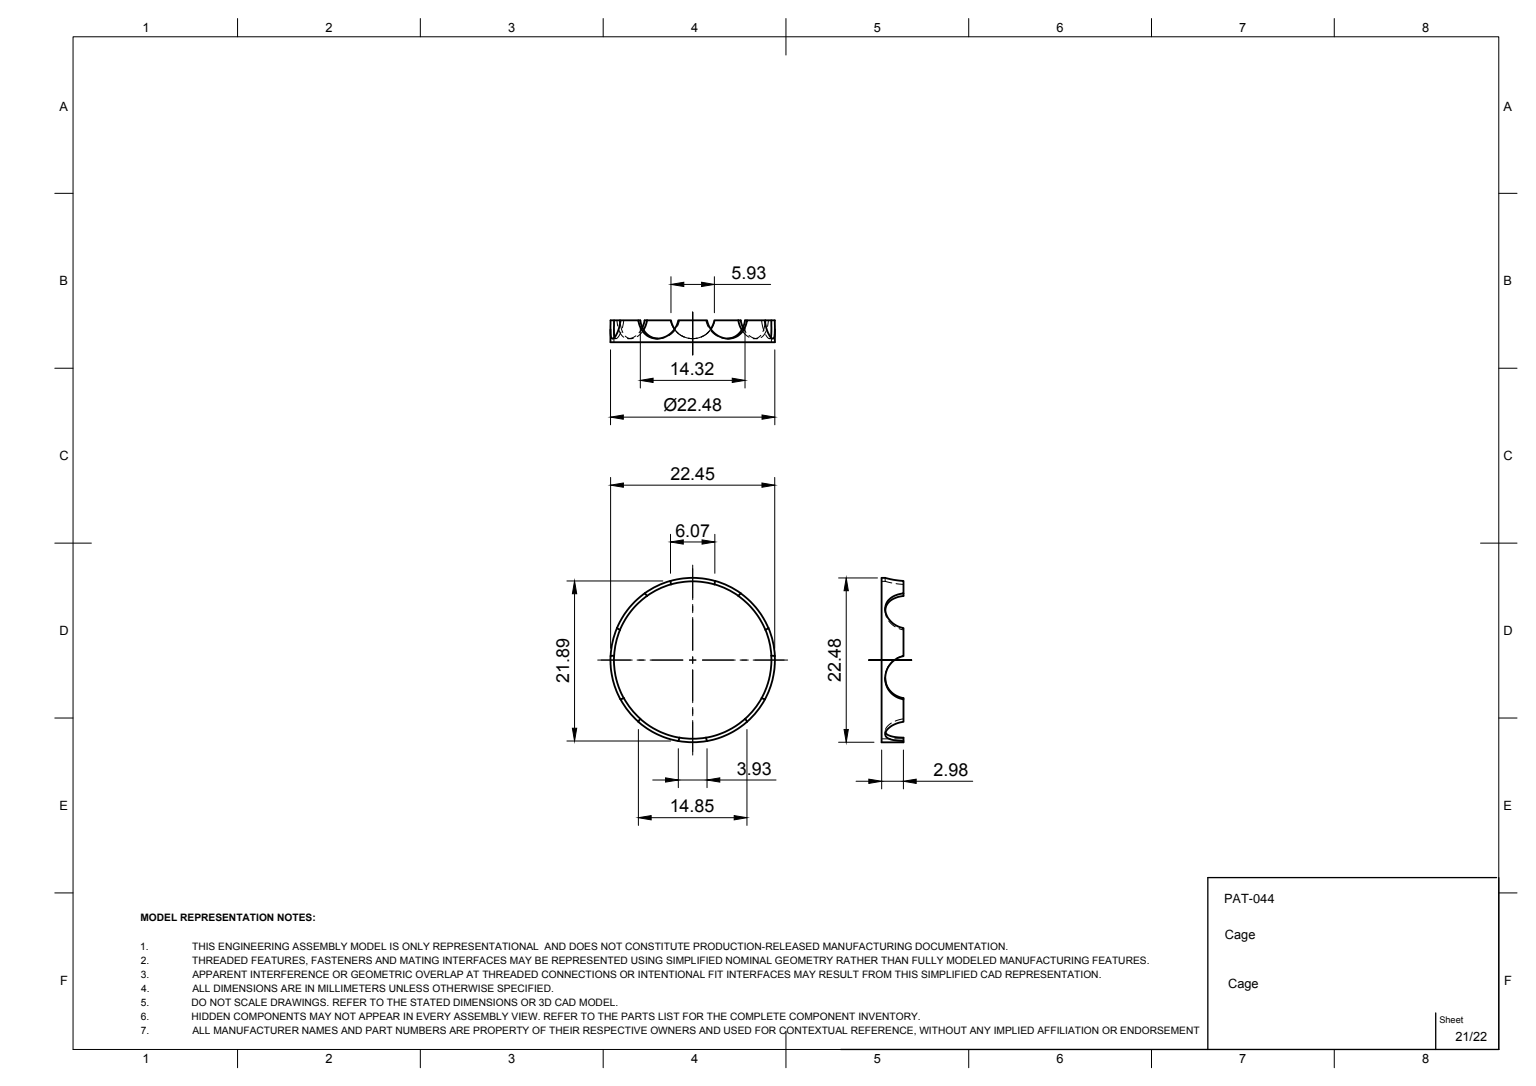
ISO-10303-21;
HEADER;
/* Generated by software containing ST-Developer
 * from STEP Tools, Inc. (www.steptools.com) 
 */

FILE_DESCRIPTION(
/* description */ ('Four-wheel beam trolley'),
/* implementation_level */ '2;1');

FILE_NAME(
/* name */ 'Cage.step',
/* time_stamp */ '2026-10-29T16:22:06-07:00',
/* author */ (''),
/* organization */ (''),
/* preprocessor_version */ 'ST-DEVELOPER v20.2',
/* originating_system */ 'Autodesk Translation Framework v15.17.0.0',
/* authorisation */ '');

FILE_SCHEMA (('AUTOMOTIVE_DESIGN { 1 0 10303 214 3 1 1 }'));
ENDSEC;

DATA;
#10=MECHANICAL_DESIGN_GEOMETRIC_PRESENTATION_REPRESENTATION('',(#298),#4777);
#11=B_SPLINE_CURVE_WITH_KNOTS('',3,(#4287,#4288,#4289,#4290,#4291,#4292,
#4293,#4294,#4295,#4296,#4297,#4298,#4299,#4300,#4301,#4302,#4303,#4304,
#4305,#4306,#4307,#4308),.UNSPECIFIED.,.F.,.F.,(4,2,2,2,2,2,2,2,2,2,4),
(0.0591825211272536,0.157966726598481,0.236950089897721,0.315933453196962,
0.391576304923761,0.46721915665056,0.54286200837736,0.618504860104159,0.697488223403399,
0.77647158670264,0.875255792173867),.UNSPECIFIED.);
#12=B_SPLINE_CURVE_WITH_KNOTS('',3,(#4312,#4313,#4314,#4315,#4316,#4317,
#4318,#4319,#4320,#4321,#4322,#4323,#4324,#4325,#4326,#4327,#4328,#4329,
#4330,#4331,#4332,#4333),.UNSPECIFIED.,.F.,.F.,(4,2,2,2,2,2,2,2,2,2,4),
(0.0581119756758434,0.106553146291161,0.213106292582322,0.30849933801665,
0.386091982889075,0.4636846277615,0.541277272633925,0.61886991750635,0.714262962940678,
0.820816109231839,0.869257279847157),.UNSPECIFIED.);
#13=B_SPLINE_CURVE_WITH_KNOTS('',3,(#4339,#4340,#4341,#4342,#4343,#4344,
#4345,#4346,#4347,#4348,#4349,#4350,#4351,#4352,#4353,#4354,#4355,#4356,
#4357,#4358,#4359,#4360),.UNSPECIFIED.,.F.,.F.,(4,2,2,2,2,2,2,2,2,2,4),
(0.0581119756758434,0.106553146291161,0.213106292582322,0.30849933801665,
0.386091982889075,0.4636846277615,0.541277272633925,0.61886991750635,0.714262962940679,
0.820816109231839,0.869257279847157),.UNSPECIFIED.);
#14=B_SPLINE_CURVE_WITH_KNOTS('',3,(#4364,#4365,#4366,#4367,#4368,#4369,
#4370,#4371,#4372,#4373,#4374,#4375,#4376,#4377,#4378,#4379,#4380,#4381,
#4382,#4383,#4384,#4385),.UNSPECIFIED.,.F.,.F.,(4,2,2,2,2,2,2,2,2,2,4),
(0.0581119756758433,0.106553146291161,0.213106292582322,0.308499338016649,
0.386091982889075,0.4636846277615,0.541277272633925,0.61886991750635,0.714262962940678,
0.820816109231839,0.869257279847157),.UNSPECIFIED.);
#15=B_SPLINE_CURVE_WITH_KNOTS('',3,(#4394,#4395,#4396,#4397,#4398,#4399,
#4400,#4401,#4402,#4403,#4404,#4405,#4406,#4407,#4408,#4409,#4410,#4411,
#4412,#4413,#4414,#4415),.UNSPECIFIED.,.F.,.F.,(4,2,2,2,2,2,2,2,2,2,4),
(0.0581119756758433,0.106553146291161,0.213106292582322,0.30849933801665,
0.386091982889075,0.4636846277615,0.541277272633925,0.61886991750635,0.714262962940678,
0.820816109231839,0.869257279847157),.UNSPECIFIED.);
#16=B_SPLINE_CURVE_WITH_KNOTS('',3,(#4419,#4420,#4421,#4422,#4423,#4424,
#4425,#4426,#4427,#4428,#4429,#4430,#4431,#4432,#4433,#4434,#4435,#4436,
#4437,#4438,#4439,#4440),.UNSPECIFIED.,.F.,.F.,(4,2,2,2,2,2,2,2,2,2,4),
(0.0581119756758434,0.106553146291161,0.213106292582322,0.30849933801665,
0.386091982889075,0.4636846277615,0.541277272633925,0.61886991750635,0.714262962940678,
0.820816109231839,0.869257279847157),.UNSPECIFIED.);
#17=B_SPLINE_CURVE_WITH_KNOTS('',3,(#4444,#4445,#4446,#4447,#4448,#4449,
#4450,#4451,#4452,#4453,#4454,#4455,#4456,#4457,#4458,#4459,#4460,#4461,
#4462,#4463,#4464,#4465),.UNSPECIFIED.,.F.,.F.,(4,2,2,2,2,2,2,2,2,2,4),
(0.0581119756758434,0.106553146291161,0.213106292582322,0.30849933801665,
0.386091982889075,0.4636846277615,0.541277272633925,0.61886991750635,0.714262962940678,
0.820816109231839,0.869257279847157),.UNSPECIFIED.);
#18=B_SPLINE_CURVE_WITH_KNOTS('',3,(#4469,#4470,#4471,#4472,#4473,#4474,
#4475,#4476,#4477,#4478,#4479,#4480,#4481,#4482,#4483,#4484,#4485,#4486,
#4487,#4488,#4489,#4490),.UNSPECIFIED.,.F.,.F.,(4,2,2,2,2,2,2,2,2,2,4),
(0.0581119756758433,0.106553146291161,0.213106292582322,0.30849933801665,
0.386091982889075,0.4636846277615,0.541277272633925,0.61886991750635,0.714262962940678,
0.820816109231839,0.869257279847157),.UNSPECIFIED.);
#19=B_SPLINE_CURVE_WITH_KNOTS('',3,(#4498,#4499,#4500,#4501,#4502,#4503,
#4504,#4505,#4506,#4507,#4508,#4509,#4510,#4511,#4512,#4513,#4514,#4515,
#4516,#4517,#4518,#4519),.UNSPECIFIED.,.F.,.F.,(4,2,2,2,2,2,2,2,2,2,4),
(0.0591825211272536,0.157966726598481,0.236950089897721,0.315933453196962,
0.391576304923761,0.467219156650561,0.54286200837736,0.618504860104159,
0.697488223403399,0.77647158670264,0.875255792173867),.UNSPECIFIED.);
#20=B_SPLINE_CURVE_WITH_KNOTS('',3,(#4527,#4528,#4529,#4530,#4531,#4532,
#4533,#4534,#4535,#4536,#4537,#4538,#4539,#4540,#4541,#4542,#4543,#4544,
#4545,#4546,#4547,#4548),.UNSPECIFIED.,.F.,.F.,(4,2,2,2,2,2,2,2,2,2,4),
(0.0591825211272536,0.157966726598481,0.236950089897722,0.315933453196962,
0.391576304923761,0.467219156650561,0.54286200837736,0.618504860104159,
0.697488223403399,0.77647158670264,0.875255792173867),.UNSPECIFIED.);
#21=B_SPLINE_CURVE_WITH_KNOTS('',3,(#4558,#4559,#4560,#4561,#4562,#4563,
#4564,#4565,#4566,#4567,#4568,#4569,#4570,#4571,#4572,#4573,#4574,#4575,
#4576,#4577,#4578,#4579),.UNSPECIFIED.,.F.,.F.,(4,2,2,2,2,2,2,2,2,2,4),
(0.0591825211272536,0.157966726598481,0.236950089897721,0.315933453196962,
0.391576304923761,0.46721915665056,0.54286200837736,0.618504860104159,0.697488223403399,
0.77647158670264,0.875255792173867),.UNSPECIFIED.);
#22=B_SPLINE_CURVE_WITH_KNOTS('',3,(#4587,#4588,#4589,#4590,#4591,#4592,
#4593,#4594,#4595,#4596,#4597,#4598,#4599,#4600,#4601,#4602,#4603,#4604,
#4605,#4606,#4607,#4608),.UNSPECIFIED.,.F.,.F.,(4,2,2,2,2,2,2,2,2,2,4),
(0.0591825211272536,0.157966726598481,0.236950089897721,0.315933453196962,
0.391576304923761,0.46721915665056,0.542862008377359,0.618504860104159,
0.697488223403399,0.776471586702639,0.875255792173867),.UNSPECIFIED.);
#23=B_SPLINE_CURVE_WITH_KNOTS('',3,(#4616,#4617,#4618,#4619,#4620,#4621,
#4622,#4623,#4624,#4625,#4626,#4627,#4628,#4629,#4630,#4631,#4632,#4633,
#4634,#4635,#4636,#4637),.UNSPECIFIED.,.F.,.F.,(4,2,2,2,2,2,2,2,2,2,4),
(0.0591825211272536,0.157966726598481,0.236950089897721,0.315933453196962,
0.391576304923761,0.46721915665056,0.54286200837736,0.618504860104159,0.697488223403399,
0.77647158670264,0.875255792173867),.UNSPECIFIED.);
#24=B_SPLINE_CURVE_WITH_KNOTS('',3,(#4646,#4647,#4648,#4649,#4650,#4651,
#4652,#4653,#4654,#4655,#4656,#4657,#4658,#4659,#4660,#4661,#4662,#4663,
#4664,#4665,#4666,#4667),.UNSPECIFIED.,.F.,.F.,(4,2,2,2,2,2,2,2,2,2,4),
(0.0591825211272536,0.157966726598481,0.236950089897721,0.315933453196962,
0.391576304923761,0.46721915665056,0.542862008377359,0.618504860104159,
0.697488223403399,0.776471586702639,0.875255792173867),.UNSPECIFIED.);
#32=SPHERICAL_SURFACE('',#2842,0.309556);
#33=SPHERICAL_SURFACE('',#2858,0.309556);
#34=SPHERICAL_SURFACE('',#2863,0.309556);
#35=SPHERICAL_SURFACE('',#2869,0.309556);
#36=SPHERICAL_SURFACE('',#2874,0.309556);
#37=SPHERICAL_SURFACE('',#2879,0.309556);
#38=SPHERICAL_SURFACE('',#2887,0.309556);
#258=SHAPE_REPRESENTATION_RELATIONSHIP('SRR','None',#4889,#275);
#275=ADVANCED_BREP_SHAPE_REPRESENTATION('',(#320),#4774);
#298=STYLED_ITEM('',(#5056),#320);
#320=MANIFOLD_SOLID_BREP('Continuous crown cage',#2387);
#358=FACE_BOUND('',#757,.T.);
#428=PLANE('',#2855);
#429=PLANE('',#2860);
#430=PLANE('',#2865);
#431=PLANE('',#2871);
#432=PLANE('',#2876);
#433=PLANE('',#2885);
#434=PLANE('',#2889);
#435=PLANE('',#2890);
#560=FACE_OUTER_BOUND('',#741,.T.);
#561=FACE_OUTER_BOUND('',#742,.T.);
#562=FACE_OUTER_BOUND('',#743,.T.);
#563=FACE_OUTER_BOUND('',#744,.T.);
#564=FACE_OUTER_BOUND('',#745,.T.);
#565=FACE_OUTER_BOUND('',#746,.T.);
#566=FACE_OUTER_BOUND('',#747,.T.);
#567=FACE_OUTER_BOUND('',#748,.T.);
#568=FACE_OUTER_BOUND('',#749,.T.);
#569=FACE_OUTER_BOUND('',#750,.T.);
#570=FACE_OUTER_BOUND('',#751,.T.);
#571=FACE_OUTER_BOUND('',#752,.T.);
#572=FACE_OUTER_BOUND('',#753,.T.);
#573=FACE_OUTER_BOUND('',#754,.T.);
#574=FACE_OUTER_BOUND('',#755,.T.);
#575=FACE_OUTER_BOUND('',#756,.T.);
#576=FACE_OUTER_BOUND('',#758,.T.);
#741=EDGE_LOOP('',(#2043,#2044,#2045,#2046));
#742=EDGE_LOOP('',(#2047,#2048,#2049,#2050,#2051,#2052,#2053,#2054,#2055,
#2056,#2057,#2058,#2059,#2060,#2061,#2062,#2063,#2064));
#743=EDGE_LOOP('',(#2065,#2066,#2067,#2068));
#744=EDGE_LOOP('',(#2069,#2070,#2071,#2072));
#745=EDGE_LOOP('',(#2073,#2074,#2075,#2076));
#746=EDGE_LOOP('',(#2077,#2078,#2079,#2080));
#747=EDGE_LOOP('',(#2081,#2082,#2083,#2084,#2085,#2086));
#748=EDGE_LOOP('',(#2087,#2088,#2089,#2090));
#749=EDGE_LOOP('',(#2091,#2092,#2093,#2094));
#750=EDGE_LOOP('',(#2095,#2096,#2097,#2098));
#751=EDGE_LOOP('',(#2099,#2100,#2101,#2102));
#752=EDGE_LOOP('',(#2103,#2104,#2105,#2106));
#753=EDGE_LOOP('',(#2107,#2108,#2109,#2110,#2111,#2112,#2113,#2114,#2115,
#2116,#2117,#2118,#2119,#2120,#2121,#2122,#2123,#2124));
#754=EDGE_LOOP('',(#2125,#2126,#2127,#2128));
#755=EDGE_LOOP('',(#2129,#2130,#2131,#2132));
#756=EDGE_LOOP('',(#2133));
#757=EDGE_LOOP('',(#2134));
#758=EDGE_LOOP('',(#2135,#2136,#2137,#2138));
#892=LINE('',#4389,#1015);
#893=LINE('',#4642,#1016);
#1015=VECTOR('',#3587,1.123812);
#1016=VECTOR('',#3656,1.076188);
#1117=CIRCLE('',#2843,0.303778037777585);
#1118=CIRCLE('',#2844,0.303778037777585);
#1119=CIRCLE('',#2846,1.123812);
#1120=CIRCLE('',#2847,1.123812);
#1121=CIRCLE('',#2848,1.123812);
#1122=CIRCLE('',#2849,1.123812);
#1123=CIRCLE('',#2850,1.123812);
#1124=CIRCLE('',#2851,1.123812);
#1125=CIRCLE('',#2852,1.123812);
#1126=CIRCLE('',#2853,1.123812);
#1127=CIRCLE('',#2854,1.123812);
#1128=CIRCLE('',#2856,1.076188);
#1129=CIRCLE('',#2857,0.303778037777585);
#1130=CIRCLE('',#2859,0.303778037777585);
#1131=CIRCLE('',#2861,1.076188);
#1132=CIRCLE('',#2862,0.303778037777585);
#1133=CIRCLE('',#2864,0.303778037777585);
#1134=CIRCLE('',#2866,1.076188);
#1135=CIRCLE('',#2867,1.076188);
#1136=CIRCLE('',#2868,0.303778037777585);
#1137=CIRCLE('',#2870,0.303778037777585);
#1138=CIRCLE('',#2872,1.076188);
#1139=CIRCLE('',#2873,0.303778037777585);
#1140=CIRCLE('',#2875,0.303778037777585);
#1141=CIRCLE('',#2877,1.076188);
#1142=CIRCLE('',#2878,0.303778037777585);
#1143=CIRCLE('',#2880,0.303778037777585);
#1144=CIRCLE('',#2882,1.076188);
#1145=CIRCLE('',#2883,1.076188);
#1146=CIRCLE('',#2884,1.076188);
#1147=CIRCLE('',#2886,0.303778037777585);
#1148=CIRCLE('',#2888,0.303778037777585);
#1306=VERTEX_POINT('',#4285);
#1307=VERTEX_POINT('',#4286);
#1308=VERTEX_POINT('',#4309);
#1309=VERTEX_POINT('',#4311);
#1310=VERTEX_POINT('',#4336);
#1311=VERTEX_POINT('',#4338);
#1312=VERTEX_POINT('',#4361);
#1313=VERTEX_POINT('',#4363);
#1314=VERTEX_POINT('',#4386);
#1315=VERTEX_POINT('',#4388);
#1316=VERTEX_POINT('',#4391);
#1317=VERTEX_POINT('',#4393);
#1318=VERTEX_POINT('',#4416);
#1319=VERTEX_POINT('',#4418);
#1320=VERTEX_POINT('',#4441);
#1321=VERTEX_POINT('',#4443);
#1322=VERTEX_POINT('',#4466);
#1323=VERTEX_POINT('',#4468);
#1324=VERTEX_POINT('',#4493);
#1325=VERTEX_POINT('',#4497);
#1326=VERTEX_POINT('',#4522);
#1327=VERTEX_POINT('',#4526);
#1328=VERTEX_POINT('',#4551);
#1329=VERTEX_POINT('',#4553);
#1330=VERTEX_POINT('',#4557);
#1331=VERTEX_POINT('',#4582);
#1332=VERTEX_POINT('',#4586);
#1333=VERTEX_POINT('',#4611);
#1334=VERTEX_POINT('',#4615);
#1335=VERTEX_POINT('',#4640);
#1336=VERTEX_POINT('',#4643);
#1337=VERTEX_POINT('',#4645);
#1559=EDGE_CURVE('',#1306,#1307,#11,.T.);
#1560=EDGE_CURVE('',#1308,#1306,#1117,.T.);
#1561=EDGE_CURVE('',#1309,#1308,#12,.T.);
#1562=EDGE_CURVE('',#1307,#1309,#1118,.T.);
#1563=EDGE_CURVE('',#1310,#1308,#1119,.T.);
#1564=EDGE_CURVE('',#1310,#1311,#13,.T.);
#1565=EDGE_CURVE('',#1312,#1311,#1120,.T.);
#1566=EDGE_CURVE('',#1312,#1313,#14,.T.);
#1567=EDGE_CURVE('',#1314,#1313,#1121,.T.);
#1568=EDGE_CURVE('',#1314,#1315,#892,.T.);
#1569=EDGE_CURVE('',#1315,#1315,#1122,.T.);
#1570=EDGE_CURVE('',#1316,#1314,#1123,.T.);
#1571=EDGE_CURVE('',#1316,#1317,#15,.T.);
#1572=EDGE_CURVE('',#1318,#1317,#1124,.T.);
#1573=EDGE_CURVE('',#1318,#1319,#16,.T.);
#1574=EDGE_CURVE('',#1320,#1319,#1125,.T.);
#1575=EDGE_CURVE('',#1320,#1321,#17,.T.);
#1576=EDGE_CURVE('',#1322,#1321,#1126,.T.);
#1577=EDGE_CURVE('',#1322,#1323,#18,.T.);
#1578=EDGE_CURVE('',#1309,#1323,#1127,.T.);
#1579=EDGE_CURVE('',#1306,#1324,#1128,.T.);
#1580=EDGE_CURVE('',#1324,#1310,#1129,.T.);
#1581=EDGE_CURVE('',#1325,#1324,#19,.T.);
#1582=EDGE_CURVE('',#1311,#1325,#1130,.T.);
#1583=EDGE_CURVE('',#1325,#1326,#1131,.T.);
#1584=EDGE_CURVE('',#1326,#1312,#1132,.T.);
#1585=EDGE_CURVE('',#1327,#1326,#20,.T.);
#1586=EDGE_CURVE('',#1313,#1327,#1133,.T.);
#1587=EDGE_CURVE('',#1327,#1328,#1134,.T.);
#1588=EDGE_CURVE('',#1328,#1329,#1135,.T.);
#1589=EDGE_CURVE('',#1329,#1316,#1136,.T.);
#1590=EDGE_CURVE('',#1330,#1329,#21,.T.);
#1591=EDGE_CURVE('',#1317,#1330,#1137,.T.);
#1592=EDGE_CURVE('',#1330,#1331,#1138,.T.);
#1593=EDGE_CURVE('',#1331,#1318,#1139,.T.);
#1594=EDGE_CURVE('',#1332,#1331,#22,.T.);
#1595=EDGE_CURVE('',#1319,#1332,#1140,.T.);
#1596=EDGE_CURVE('',#1332,#1333,#1141,.T.);
#1597=EDGE_CURVE('',#1333,#1320,#1142,.T.);
#1598=EDGE_CURVE('',#1334,#1333,#23,.T.);
#1599=EDGE_CURVE('',#1321,#1334,#1143,.T.);
#1600=EDGE_CURVE('',#1335,#1335,#1144,.T.);
#1601=EDGE_CURVE('',#1335,#1328,#893,.T.);
#1602=EDGE_CURVE('',#1336,#1307,#1145,.T.);
#1603=EDGE_CURVE('',#1336,#1337,#24,.T.);
#1604=EDGE_CURVE('',#1334,#1337,#1146,.T.);
#1605=EDGE_CURVE('',#1323,#1336,#1147,.T.);
#1606=EDGE_CURVE('',#1337,#1322,#1148,.T.);
#2043=ORIENTED_EDGE('',*,*,#1559,.F.);
#2044=ORIENTED_EDGE('',*,*,#1560,.F.);
#2045=ORIENTED_EDGE('',*,*,#1561,.F.);
#2046=ORIENTED_EDGE('',*,*,#1562,.F.);
#2047=ORIENTED_EDGE('',*,*,#1561,.T.);
#2048=ORIENTED_EDGE('',*,*,#1563,.F.);
#2049=ORIENTED_EDGE('',*,*,#1564,.T.);
#2050=ORIENTED_EDGE('',*,*,#1565,.F.);
#2051=ORIENTED_EDGE('',*,*,#1566,.T.);
#2052=ORIENTED_EDGE('',*,*,#1567,.F.);
#2053=ORIENTED_EDGE('',*,*,#1568,.T.);
#2054=ORIENTED_EDGE('',*,*,#1569,.F.);
#2055=ORIENTED_EDGE('',*,*,#1568,.F.);
#2056=ORIENTED_EDGE('',*,*,#1570,.F.);
#2057=ORIENTED_EDGE('',*,*,#1571,.T.);
#2058=ORIENTED_EDGE('',*,*,#1572,.F.);
#2059=ORIENTED_EDGE('',*,*,#1573,.T.);
#2060=ORIENTED_EDGE('',*,*,#1574,.F.);
#2061=ORIENTED_EDGE('',*,*,#1575,.T.);
#2062=ORIENTED_EDGE('',*,*,#1576,.F.);
#2063=ORIENTED_EDGE('',*,*,#1577,.T.);
#2064=ORIENTED_EDGE('',*,*,#1578,.F.);
#2065=ORIENTED_EDGE('',*,*,#1560,.T.);
#2066=ORIENTED_EDGE('',*,*,#1579,.T.);
#2067=ORIENTED_EDGE('',*,*,#1580,.T.);
#2068=ORIENTED_EDGE('',*,*,#1563,.T.);
#2069=ORIENTED_EDGE('',*,*,#1581,.F.);
#2070=ORIENTED_EDGE('',*,*,#1582,.F.);
#2071=ORIENTED_EDGE('',*,*,#1564,.F.);
#2072=ORIENTED_EDGE('',*,*,#1580,.F.);
#2073=ORIENTED_EDGE('',*,*,#1582,.T.);
#2074=ORIENTED_EDGE('',*,*,#1583,.T.);
#2075=ORIENTED_EDGE('',*,*,#1584,.T.);
#2076=ORIENTED_EDGE('',*,*,#1565,.T.);
#2077=ORIENTED_EDGE('',*,*,#1585,.F.);
#2078=ORIENTED_EDGE('',*,*,#1586,.F.);
#2079=ORIENTED_EDGE('',*,*,#1566,.F.);
#2080=ORIENTED_EDGE('',*,*,#1584,.F.);
#2081=ORIENTED_EDGE('',*,*,#1586,.T.);
#2082=ORIENTED_EDGE('',*,*,#1587,.T.);
#2083=ORIENTED_EDGE('',*,*,#1588,.T.);
#2084=ORIENTED_EDGE('',*,*,#1589,.T.);
#2085=ORIENTED_EDGE('',*,*,#1570,.T.);
#2086=ORIENTED_EDGE('',*,*,#1567,.T.);
#2087=ORIENTED_EDGE('',*,*,#1590,.F.);
#2088=ORIENTED_EDGE('',*,*,#1591,.F.);
#2089=ORIENTED_EDGE('',*,*,#1571,.F.);
#2090=ORIENTED_EDGE('',*,*,#1589,.F.);
#2091=ORIENTED_EDGE('',*,*,#1591,.T.);
#2092=ORIENTED_EDGE('',*,*,#1592,.T.);
#2093=ORIENTED_EDGE('',*,*,#1593,.T.);
#2094=ORIENTED_EDGE('',*,*,#1572,.T.);
#2095=ORIENTED_EDGE('',*,*,#1594,.F.);
#2096=ORIENTED_EDGE('',*,*,#1595,.F.);
#2097=ORIENTED_EDGE('',*,*,#1573,.F.);
#2098=ORIENTED_EDGE('',*,*,#1593,.F.);
#2099=ORIENTED_EDGE('',*,*,#1595,.T.);
#2100=ORIENTED_EDGE('',*,*,#1596,.T.);
#2101=ORIENTED_EDGE('',*,*,#1597,.T.);
#2102=ORIENTED_EDGE('',*,*,#1574,.T.);
#2103=ORIENTED_EDGE('',*,*,#1575,.F.);
#2104=ORIENTED_EDGE('',*,*,#1597,.F.);
#2105=ORIENTED_EDGE('',*,*,#1598,.F.);
#2106=ORIENTED_EDGE('',*,*,#1599,.F.);
#2107=ORIENTED_EDGE('',*,*,#1600,.F.);
#2108=ORIENTED_EDGE('',*,*,#1601,.T.);
#2109=ORIENTED_EDGE('',*,*,#1587,.F.);
#2110=ORIENTED_EDGE('',*,*,#1585,.T.);
#2111=ORIENTED_EDGE('',*,*,#1583,.F.);
#2112=ORIENTED_EDGE('',*,*,#1581,.T.);
#2113=ORIENTED_EDGE('',*,*,#1579,.F.);
#2114=ORIENTED_EDGE('',*,*,#1559,.T.);
#2115=ORIENTED_EDGE('',*,*,#1602,.F.);
#2116=ORIENTED_EDGE('',*,*,#1603,.T.);
#2117=ORIENTED_EDGE('',*,*,#1604,.F.);
#2118=ORIENTED_EDGE('',*,*,#1598,.T.);
#2119=ORIENTED_EDGE('',*,*,#1596,.F.);
#2120=ORIENTED_EDGE('',*,*,#1594,.T.);
#2121=ORIENTED_EDGE('',*,*,#1592,.F.);
#2122=ORIENTED_EDGE('',*,*,#1590,.T.);
#2123=ORIENTED_EDGE('',*,*,#1588,.F.);
#2124=ORIENTED_EDGE('',*,*,#1601,.F.);
#2125=ORIENTED_EDGE('',*,*,#1562,.T.);
#2126=ORIENTED_EDGE('',*,*,#1578,.T.);
#2127=ORIENTED_EDGE('',*,*,#1605,.T.);
#2128=ORIENTED_EDGE('',*,*,#1602,.T.);
#2129=ORIENTED_EDGE('',*,*,#1577,.F.);
#2130=ORIENTED_EDGE('',*,*,#1606,.F.);
#2131=ORIENTED_EDGE('',*,*,#1603,.F.);
#2132=ORIENTED_EDGE('',*,*,#1605,.F.);
#2133=ORIENTED_EDGE('',*,*,#1569,.T.);
#2134=ORIENTED_EDGE('',*,*,#1600,.T.);
#2135=ORIENTED_EDGE('',*,*,#1599,.T.);
#2136=ORIENTED_EDGE('',*,*,#1604,.T.);
#2137=ORIENTED_EDGE('',*,*,#1606,.T.);
#2138=ORIENTED_EDGE('',*,*,#1576,.T.);
#2210=CYLINDRICAL_SURFACE('',#2845,1.123812);
#2211=CYLINDRICAL_SURFACE('',#2881,1.076188);
#2336=ADVANCED_FACE('',(#560),#32,.F.);
#2337=ADVANCED_FACE('',(#561),#2210,.T.);
#2338=ADVANCED_FACE('',(#562),#428,.T.);
#2339=ADVANCED_FACE('',(#563),#33,.F.);
#2340=ADVANCED_FACE('',(#564),#429,.T.);
#2341=ADVANCED_FACE('',(#565),#34,.F.);
#2342=ADVANCED_FACE('',(#566),#430,.T.);
#2343=ADVANCED_FACE('',(#567),#35,.F.);
#2344=ADVANCED_FACE('',(#568),#431,.T.);
#2345=ADVANCED_FACE('',(#569),#36,.F.);
#2346=ADVANCED_FACE('',(#570),#432,.T.);
#2347=ADVANCED_FACE('',(#571),#37,.F.);
#2348=ADVANCED_FACE('',(#572),#2211,.F.);
#2349=ADVANCED_FACE('',(#573),#433,.T.);
#2350=ADVANCED_FACE('',(#574),#38,.F.);
#2351=ADVANCED_FACE('',(#575,#358),#434,.T.);
#2352=ADVANCED_FACE('',(#576),#435,.T.);
#2387=CLOSED_SHELL('',(#2336,#2337,#2338,#2339,#2340,#2341,#2342,#2343,
#2344,#2345,#2346,#2347,#2348,#2349,#2350,#2351,#2352));
#2841=AXIS2_PLACEMENT_3D('',#4283,#3571,#3572);
#2842=AXIS2_PLACEMENT_3D('',#4284,#3573,#3574);
#2843=AXIS2_PLACEMENT_3D('',#4310,#3575,#3576);
#2844=AXIS2_PLACEMENT_3D('',#4334,#3577,#3578);
#2845=AXIS2_PLACEMENT_3D('',#4335,#3579,#3580);
#2846=AXIS2_PLACEMENT_3D('',#4337,#3581,#3582);
#2847=AXIS2_PLACEMENT_3D('',#4362,#3583,#3584);
#2848=AXIS2_PLACEMENT_3D('',#4387,#3585,#3586);
#2849=AXIS2_PLACEMENT_3D('',#4390,#3588,#3589);
#2850=AXIS2_PLACEMENT_3D('',#4392,#3590,#3591);
#2851=AXIS2_PLACEMENT_3D('',#4417,#3592,#3593);
#2852=AXIS2_PLACEMENT_3D('',#4442,#3594,#3595);
#2853=AXIS2_PLACEMENT_3D('',#4467,#3596,#3597);
#2854=AXIS2_PLACEMENT_3D('',#4491,#3598,#3599);
#2855=AXIS2_PLACEMENT_3D('',#4492,#3600,#3601);
#2856=AXIS2_PLACEMENT_3D('',#4494,#3602,#3603);
#2857=AXIS2_PLACEMENT_3D('',#4495,#3604,#3605);
#2858=AXIS2_PLACEMENT_3D('',#4496,#3606,#3607);
#2859=AXIS2_PLACEMENT_3D('',#4520,#3608,#3609);
#2860=AXIS2_PLACEMENT_3D('',#4521,#3610,#3611);
#2861=AXIS2_PLACEMENT_3D('',#4523,#3612,#3613);
#2862=AXIS2_PLACEMENT_3D('',#4524,#3614,#3615);
#2863=AXIS2_PLACEMENT_3D('',#4525,#3616,#3617);
#2864=AXIS2_PLACEMENT_3D('',#4549,#3618,#3619);
#2865=AXIS2_PLACEMENT_3D('',#4550,#3620,#3621);
#2866=AXIS2_PLACEMENT_3D('',#4552,#3622,#3623);
#2867=AXIS2_PLACEMENT_3D('',#4554,#3624,#3625);
#2868=AXIS2_PLACEMENT_3D('',#4555,#3626,#3627);
#2869=AXIS2_PLACEMENT_3D('',#4556,#3628,#3629);
#2870=AXIS2_PLACEMENT_3D('',#4580,#3630,#3631);
#2871=AXIS2_PLACEMENT_3D('',#4581,#3632,#3633);
#2872=AXIS2_PLACEMENT_3D('',#4583,#3634,#3635);
#2873=AXIS2_PLACEMENT_3D('',#4584,#3636,#3637);
#2874=AXIS2_PLACEMENT_3D('',#4585,#3638,#3639);
#2875=AXIS2_PLACEMENT_3D('',#4609,#3640,#3641);
#2876=AXIS2_PLACEMENT_3D('',#4610,#3642,#3643);
#2877=AXIS2_PLACEMENT_3D('',#4612,#3644,#3645);
#2878=AXIS2_PLACEMENT_3D('',#4613,#3646,#3647);
#2879=AXIS2_PLACEMENT_3D('',#4614,#3648,#3649);
#2880=AXIS2_PLACEMENT_3D('',#4638,#3650,#3651);
#2881=AXIS2_PLACEMENT_3D('',#4639,#3652,#3653);
#2882=AXIS2_PLACEMENT_3D('',#4641,#3654,#3655);
#2883=AXIS2_PLACEMENT_3D('',#4644,#3657,#3658);
#2884=AXIS2_PLACEMENT_3D('',#4668,#3659,#3660);
#2885=AXIS2_PLACEMENT_3D('',#4669,#3661,#3662);
#2886=AXIS2_PLACEMENT_3D('',#4670,#3663,#3664);
#2887=AXIS2_PLACEMENT_3D('',#4671,#3665,#3666);
#2888=AXIS2_PLACEMENT_3D('',#4672,#3667,#3668);
#2889=AXIS2_PLACEMENT_3D('',#4673,#3669,#3670);
#2890=AXIS2_PLACEMENT_3D('',#4674,#3671,#3672);
#3571=DIRECTION('axis',(0.,0.,1.));
#3572=DIRECTION('refdir',(1.,0.,0.));
#3573=DIRECTION('center_axis',(0.,0.,1.));
#3574=DIRECTION('ref_axis',(1.,0.,0.));
#3575=DIRECTION('center_axis',(0.,-1.,0.));
#3576=DIRECTION('ref_axis',(0.,0.,-1.));
#3577=DIRECTION('center_axis',(0.,-1.,0.));
#3578=DIRECTION('ref_axis',(0.,0.,-1.));
#3579=DIRECTION('center_axis',(0.,1.,0.));
#3580=DIRECTION('ref_axis',(1.,0.,0.));
#3581=DIRECTION('center_axis',(0.,1.,0.));
#3582=DIRECTION('ref_axis',(1.,0.,0.));
#3583=DIRECTION('center_axis',(0.,1.,0.));
#3584=DIRECTION('ref_axis',(1.,0.,0.));
#3585=DIRECTION('center_axis',(0.,1.,0.));
#3586=DIRECTION('ref_axis',(1.,0.,0.));
#3587=DIRECTION('',(0.,-1.,0.));
#3588=DIRECTION('center_axis',(0.,-1.,0.));
#3589=DIRECTION('ref_axis',(1.,0.,0.));
#3590=DIRECTION('center_axis',(0.,1.,0.));
#3591=DIRECTION('ref_axis',(1.,0.,0.));
#3592=DIRECTION('center_axis',(0.,1.,0.));
#3593=DIRECTION('ref_axis',(1.,0.,0.));
#3594=DIRECTION('center_axis',(0.,1.,0.));
#3595=DIRECTION('ref_axis',(1.,0.,0.));
#3596=DIRECTION('center_axis',(0.,1.,0.));
#3597=DIRECTION('ref_axis',(1.,0.,0.));
#3598=DIRECTION('center_axis',(0.,1.,0.));
#3599=DIRECTION('ref_axis',(1.,0.,0.));
#3600=DIRECTION('center_axis',(0.,1.,0.));
#3601=DIRECTION('ref_axis',(1.,0.,0.));
#3602=DIRECTION('center_axis',(0.,-1.,0.));
#3603=DIRECTION('ref_axis',(1.,0.,0.));
#3604=DIRECTION('center_axis',(0.,-1.,0.));
#3605=DIRECTION('ref_axis',(0.,0.,-1.));
#3606=DIRECTION('center_axis',(8.96625347776458E-17,0.,1.));
#3607=DIRECTION('ref_axis',(1.,0.,0.));
#3608=DIRECTION('center_axis',(0.,-1.,0.));
#3609=DIRECTION('ref_axis',(0.,0.,-1.));
#3610=DIRECTION('center_axis',(0.,1.,0.));
#3611=DIRECTION('ref_axis',(1.,0.,0.));
#3612=DIRECTION('center_axis',(0.,-1.,0.));
#3613=DIRECTION('ref_axis',(1.,0.,0.));
#3614=DIRECTION('center_axis',(0.,-1.,0.));
#3615=DIRECTION('ref_axis',(0.,0.,-1.));
#3616=DIRECTION('center_axis',(0.,0.,1.));
#3617=DIRECTION('ref_axis',(1.,0.,0.));
#3618=DIRECTION('center_axis',(0.,-1.,0.));
#3619=DIRECTION('ref_axis',(0.,0.,-1.));
#3620=DIRECTION('center_axis',(0.,1.,0.));
#3621=DIRECTION('ref_axis',(1.,0.,0.));
#3622=DIRECTION('center_axis',(0.,-1.,0.));
#3623=DIRECTION('ref_axis',(1.,0.,0.));
#3624=DIRECTION('center_axis',(0.,-1.,0.));
#3625=DIRECTION('ref_axis',(1.,0.,0.));
#3626=DIRECTION('center_axis',(0.,-1.,0.));
#3627=DIRECTION('ref_axis',(0.,0.,-1.));
#3628=DIRECTION('center_axis',(0.,0.,1.));
#3629=DIRECTION('ref_axis',(1.,0.,0.));
#3630=DIRECTION('center_axis',(0.,-1.,0.));
#3631=DIRECTION('ref_axis',(0.,0.,-1.));
#3632=DIRECTION('center_axis',(0.,1.,0.));
#3633=DIRECTION('ref_axis',(1.,0.,0.));
#3634=DIRECTION('center_axis',(0.,-1.,0.));
#3635=DIRECTION('ref_axis',(1.,0.,0.));
#3636=DIRECTION('center_axis',(0.,-1.,0.));
#3637=DIRECTION('ref_axis',(0.,0.,-1.));
#3638=DIRECTION('center_axis',(8.96625347776458E-17,0.,1.));
#3639=DIRECTION('ref_axis',(1.,0.,0.));
#3640=DIRECTION('center_axis',(0.,-1.,0.));
#3641=DIRECTION('ref_axis',(0.,0.,-1.));
#3642=DIRECTION('center_axis',(0.,1.,0.));
#3643=DIRECTION('ref_axis',(1.,0.,0.));
#3644=DIRECTION('center_axis',(0.,-1.,0.));
#3645=DIRECTION('ref_axis',(1.,0.,0.));
#3646=DIRECTION('center_axis',(0.,-1.,0.));
#3647=DIRECTION('ref_axis',(0.,0.,-1.));
#3648=DIRECTION('center_axis',(0.,0.,1.));
#3649=DIRECTION('ref_axis',(1.,0.,0.));
#3650=DIRECTION('center_axis',(0.,-1.,0.));
#3651=DIRECTION('ref_axis',(0.,0.,-1.));
#3652=DIRECTION('center_axis',(0.,1.,0.));
#3653=DIRECTION('ref_axis',(1.,0.,0.));
#3654=DIRECTION('center_axis',(0.,1.,0.));
#3655=DIRECTION('ref_axis',(1.,0.,0.));
#3656=DIRECTION('',(0.,1.,0.));
#3657=DIRECTION('center_axis',(0.,-1.,0.));
#3658=DIRECTION('ref_axis',(1.,0.,0.));
#3659=DIRECTION('center_axis',(0.,-1.,0.));
#3660=DIRECTION('ref_axis',(1.,0.,0.));
#3661=DIRECTION('center_axis',(0.,1.,0.));
#3662=DIRECTION('ref_axis',(1.,0.,0.));
#3663=DIRECTION('center_axis',(0.,-1.,0.));
#3664=DIRECTION('ref_axis',(0.,0.,-1.));
#3665=DIRECTION('center_axis',(0.,0.,1.));
#3666=DIRECTION('ref_axis',(1.,0.,0.));
#3667=DIRECTION('center_axis',(0.,-1.,0.));
#3668=DIRECTION('ref_axis',(0.,0.,-1.));
#3669=DIRECTION('center_axis',(0.,-1.,0.));
#3670=DIRECTION('ref_axis',(-1.,0.,0.));
#3671=DIRECTION('center_axis',(0.,1.,0.));
#3672=DIRECTION('ref_axis',(1.,0.,0.));
#4283=CARTESIAN_POINT('',(0.,0.,0.));
#4284=CARTESIAN_POINT('Origin',(0.685838782044607,0.,0.860014630714833));
#4285=CARTESIAN_POINT('',(0.413083465285518,-0.05953,0.993751811093549));
#4286=CARTESIAN_POINT('',(0.876916659919095,-0.05953,0.623857181492959));
#4287=CARTESIAN_POINT('Ctrl Pts',(0.413083465285518,-0.05953,0.993751811093549));
#4288=CARTESIAN_POINT('Ctrl Pts',(0.419070565453383,-0.0925528133349865,
0.991263089003441));
#4289=CARTESIAN_POINT('Ctrl Pts',(0.430199341854858,-0.124911173756694,
0.986608710139579));
#4290=CARTESIAN_POINT('Ctrl Pts',(0.457978755888596,-0.177924977804098,
0.973971221090534));
#4291=CARTESIAN_POINT('Ctrl Pts',(0.473077587363685,-0.199697230012983,
0.966820759530997));
#4292=CARTESIAN_POINT('Ctrl Pts',(0.507057380724533,-0.237895043532788,
0.949440676105255));
#4293=CARTESIAN_POINT('Ctrl Pts',(0.525933334162555,-0.254319232363049,
0.939198248544428));
#4294=CARTESIAN_POINT('Ctrl Pts',(0.564362943424238,-0.28018331644634,0.916597376014514));
#4295=CARTESIAN_POINT('Ctrl Pts',(0.585840553788742,-0.29104845371857,0.903141581680914));
#4296=CARTESIAN_POINT('Ctrl Pts',(0.629305439856167,-0.30527573347708,0.873412008702649));
#4297=CARTESIAN_POINT('Ctrl Pts',(0.651278921914856,-0.308638795020976,
0.857118508332695));
#4298=CARTESIAN_POINT('Ctrl Pts',(0.690705563850638,-0.308638795020976,
0.825676810575914));
#4299=CARTESIAN_POINT('Ctrl Pts',(0.711480111898423,-0.30527573347708,0.807879894508811));
#4300=CARTESIAN_POINT('Ctrl Pts',(0.750136149454208,-0.29104845371857,0.772120216227122));
#4301=CARTESIAN_POINT('Ctrl Pts',(0.768033796848072,-0.28018331644634,0.754175290318038));
#4302=CARTESIAN_POINT('Ctrl Pts',(0.798619410861634,-0.254319232363049,
0.721738358858166));
#4303=CARTESIAN_POINT('Ctrl Pts',(0.812805334167529,-0.237895043532788,
0.705614819529209));
#4304=CARTESIAN_POINT('Ctrl Pts',(0.837310877969633,-0.199697230012983,
0.676354402927683));
#4305=CARTESIAN_POINT('Ctrl Pts',(0.847641868610495,-0.177924977804098,
0.663225258065736));
#4306=CARTESIAN_POINT('Ctrl Pts',(0.866144010579847,-0.124911173756694,
0.638954437806245));
#4307=CARTESIAN_POINT('Ctrl Pts',(0.873158080166742,-0.0925528133349865,
0.62914037979579));
#4308=CARTESIAN_POINT('Ctrl Pts',(0.876916659919095,-0.05953,0.623857181492959));
#4309=CARTESIAN_POINT('',(0.437601487681057,-0.05953,1.03511272300331));
#4310=CARTESIAN_POINT('Origin',(0.685838782044607,-0.05953,0.860014630714833));
#4311=CARTESIAN_POINT('',(0.911784794170997,-0.05953,0.656964154625313));
#4312=CARTESIAN_POINT('Ctrl Pts',(0.911784794170998,-0.0595300000000001,
0.656964154625312));
#4313=CARTESIAN_POINT('Ctrl Pts',(0.909827729890942,-0.0762225747374255,
0.659680317203144));
#4314=CARTESIAN_POINT('Ctrl Pts',(0.907004864562642,-0.0928409665394228,
0.663576540841106));
#4315=CARTESIAN_POINT('Ctrl Pts',(0.895234408667242,-0.144299303100741,
0.679480524217551));
#4316=CARTESIAN_POINT('Ctrl Pts',(0.882797231409153,-0.177024326825049,
0.695831250979106));
#4317=CARTESIAN_POINT('Ctrl Pts',(0.854332839576145,-0.227269801620064,
0.73042219438957));
#4318=CARTESIAN_POINT('Ctrl Pts',(0.834863020612702,-0.251265615809407,
0.752807465209441));
#4319=CARTESIAN_POINT('Ctrl Pts',(0.800439809856111,-0.279889827963178,
0.789147407129766));
#4320=CARTESIAN_POINT('Ctrl Pts',(0.781998747691871,-0.290879136862659,
0.80756613568454));
#4321=CARTESIAN_POINT('Ctrl Pts',(0.742239891936898,-0.305251990234487,
0.844254137480382));
#4322=CARTESIAN_POINT('Ctrl Pts',(0.720906778729541,-0.308638795020976,
0.862505527716294));
#4323=CARTESIAN_POINT('Ctrl Pts',(0.680463863683392,-0.308638795020976,
0.894757676234429));
#4324=CARTESIAN_POINT('Ctrl Pts',(0.657923009631182,-0.305251990234488,
0.91149460735272));
#4325=CARTESIAN_POINT('Ctrl Pts',(0.613307674922609,-0.290879136862659,
0.942092777160053));
#4326=CARTESIAN_POINT('Ctrl Pts',(0.591247219971725,-0.279889827963178,
0.955972930713954));
#4327=CARTESIAN_POINT('Ctrl Pts',(0.548158511259202,-0.251265615809407,
0.981446681891443));
#4328=CARTESIAN_POINT('Ctrl Pts',(0.522002043615455,-0.227269801620063,
0.995447160474328));
#4329=CARTESIAN_POINT('Ctrl Pts',(0.481944444320713,-0.177024326825049,
1.01550068154148));
#4330=CARTESIAN_POINT('Ctrl Pts',(0.463236132117164,-0.14429930310074,1.0239876538093));
#4331=CARTESIAN_POINT('Ctrl Pts',(0.445111721969657,-0.0928409665394226,
1.03192403056628));
#4332=CARTESIAN_POINT('Ctrl Pts',(0.440685038163619,-0.0762225747374254,
1.03380912944435));
#4333=CARTESIAN_POINT('Ctrl Pts',(0.437601487681056,-0.05953,1.03511272300331));
#4334=CARTESIAN_POINT('Origin',(0.685838782044607,-0.05953,0.860014630714833));
#4335=CARTESIAN_POINT('Origin',(0.,-0.208355,0.));
#4336=CARTESIAN_POINT('',(0.0548532617164168,-0.05953,1.12247250791415));
#4337=CARTESIAN_POINT('Origin',(0.,-0.05953,0.));
#4338=CARTESIAN_POINT('',(-0.536443649899848,-0.05953,0.987512846410683));
#4339=CARTESIAN_POINT('Ctrl Pts',(0.0548532617164173,-0.0595300000000001,
1.12247250791414));
#4340=CARTESIAN_POINT('Ctrl Pts',(0.05150947068137,-0.0762225747374254,
1.12263591311425));
#4341=CARTESIAN_POINT('Ctrl Pts',(0.0467032526342597,-0.0928409665394227,
1.12285816383385));
#4342=CARTESIAN_POINT('Ctrl Pts',(0.0269302585198975,-0.144299303100741,
1.12357162229597));
#4343=CARTESIAN_POINT('Ctrl Pts',(0.006392292392153,-0.177024326825049,
1.12404235695137));
#4344=CARTESIAN_POINT('Ctrl Pts',(-0.0383992541984087,-0.227269801620063,
1.12335509974011));
#4345=CARTESIAN_POINT('Ctrl Pts',(-0.0680399972366993,-0.251265615809407,
1.12208997038458));
#4346=CARTESIAN_POINT('Ctrl Pts',(-0.117914228755037,-0.279889827963178,
1.1178344036749));
#4347=CARTESIAN_POINT('Ctrl Pts',(-0.14381238480104,-0.290879136862659,
1.11490049012186));
#4348=CARTESIAN_POINT('Ctrl Pts',(-0.19728546073067,-0.305251990234488,
1.10669035995599));
#4349=CARTESIAN_POINT('Ctrl Pts',(-0.224855950742601,-0.308638795020976,
1.10139101611326));
#4350=CARTESIAN_POINT('Ctrl Pts',(-0.275287440920027,-0.308638795020976,
1.0898803575765));
#4351=CARTESIAN_POINT('Ctrl Pts',(-0.302426893214945,-0.305251990234488,
1.08269251410343));
#4352=CARTESIAN_POINT('Ctrl Pts',(-0.35416671187353,-0.290879136862659,
1.06688848765783));
#4353=CARTESIAN_POINT('Ctrl Pts',(-0.3787731215897,-0.279889827963178,1.05829506364875));
#4354=CARTESIAN_POINT('Ctrl Pts',(-0.425554672694338,-0.251265615809407,
1.04048957871266));
#4355=CARTESIAN_POINT('Ctrl Pts',(-0.452808978448581,-0.227269801620063,
1.02876878445619));
#4356=CARTESIAN_POINT('Ctrl Pts',(-0.493462957200432,-0.177024326825049,
1.0099536580922));
#4357=CARTESIAN_POINT('Ctrl Pts',(-0.511762781179148,-0.14429930310074,
1.00061845128527));
#4358=CARTESIAN_POINT('Ctrl Pts',(-0.529268075276157,-0.0928409665394226,
0.991396466802468));
#4359=CARTESIAN_POINT('Ctrl Pts',(-0.533501897135713,-0.0762225747374254,
0.989110885965947));
#4360=CARTESIAN_POINT('Ctrl Pts',(-0.536443649899848,-0.0595300000000001,
0.987512846410683));
#4361=CARTESIAN_POINT('',(-0.843383895613249,-0.05953,0.742736168477219));
#4362=CARTESIAN_POINT('Origin',(0.,-0.05953,0.));
#4363=CARTESIAN_POINT('',(-1.10653577764992,-0.05953,0.196295654879792));
#4364=CARTESIAN_POINT('Ctrl Pts',(-0.843383895613249,-0.0595300000000001,
0.742736168477219));
#4365=CARTESIAN_POINT('Ctrl Pts',(-0.84559647055299,-0.0762225747374255,
0.740223768851062));
#4366=CARTESIAN_POINT('Ctrl Pts',(-0.848766861100456,-0.0928409665394227,
0.736604687327351));
#4367=CARTESIAN_POINT('Ctrl Pts',(-0.861652925570091,-0.144299303100741,
0.721590372101268));
#4368=CARTESIAN_POINT('Ctrl Pts',(-0.87482617317514,-0.177024326825049,
0.705826641853758));
#4369=CARTESIAN_POINT('Ctrl Pts',(-0.902215926359523,-0.227269801620063,
0.670378702718353));
#4370=CARTESIAN_POINT('Ctrl Pts',(-0.919707509403859,-0.251265615809407,
0.646415841396062));
#4371=CARTESIAN_POINT('Ctrl Pts',(-0.947476448101718,-0.279889827963178,
0.604769294586516));
#4372=CARTESIAN_POINT('Ctrl Pts',(-0.961329858300736,-0.290879136862659,
0.582692035672022));
#4373=CARTESIAN_POINT('Ctrl Pts',(-0.988250837578047,-0.305251990234488,
0.535766169015486));
#4374=CARTESIAN_POINT('Ctrl Pts',(-1.00129756308006,-0.308638795020976,
0.510906605094603));
#4375=CARTESIAN_POINT('Ctrl Pts',(-1.02374168767024,-0.308638795020976,
0.46430090015576));
#4376=CARTESIAN_POINT('Ctrl Pts',(-1.03504317708586,-0.305251990234488,
0.438600874831839));
#4377=CARTESIAN_POINT('Ctrl Pts',(-1.05494634094458,-0.290879136862659,
0.388295406390235));
#4378=CARTESIAN_POINT('Ctrl Pts',(-1.06356957703048,-0.279889827963178,
0.363699428370917));
#4379=CARTESIAN_POINT('Ctrl Pts',(-1.0788165083757,-0.251265615809407,0.316022600643821));
#4380=CARTESIAN_POINT('Ctrl Pts',(-1.08664560412098,-0.227269801620063,
0.287406530683752));
#4381=CARTESIAN_POINT('Ctrl Pts',(-1.09728268713976,-0.177024326825049,
0.243890930799337));
#4382=CARTESIAN_POINT('Ctrl Pts',(-1.10139388218929,-0.144299303100741,
0.22376314604679));
#4383=CARTESIAN_POINT('Ctrl Pts',(-1.10509821673782,-0.0928409665394227,
0.204327142733961));
#4384=CARTESIAN_POINT('Ctrl Pts',(-1.10595102243643,-0.0762225747374254,
0.199591971170104));
#4385=CARTESIAN_POINT('Ctrl Pts',(-1.10653577764992,-0.0595300000000001,
0.196295654879792));
#4386=CARTESIAN_POINT('',(-1.123812,-0.05953,1.37627276864339E-16));
#4387=CARTESIAN_POINT('Origin',(0.,-0.05953,0.));
#4388=CARTESIAN_POINT('',(-1.123812,-0.35718,1.37627276864339E-16));
#4389=CARTESIAN_POINT('',(-1.123812,-0.208355,1.37627276864339E-16));
#4390=CARTESIAN_POINT('Origin',(0.,-0.35718,0.));
#4391=CARTESIAN_POINT('',(-1.10653577764992,-0.05953,-0.196295654879793));
#4392=CARTESIAN_POINT('Origin',(0.,-0.05953,0.));
#4393=CARTESIAN_POINT('',(-0.843383895613249,-0.05953,-0.742736168477219));
#4394=CARTESIAN_POINT('Ctrl Pts',(-1.10653577764992,-0.0595300000000001,
-0.196295654879792));
#4395=CARTESIAN_POINT('Ctrl Pts',(-1.10595102243643,-0.0762225747374255,
-0.199591971170104));
#4396=CARTESIAN_POINT('Ctrl Pts',(-1.10509821673782,-0.0928409665394228,
-0.204327142733962));
#4397=CARTESIAN_POINT('Ctrl Pts',(-1.10139388218929,-0.144299303100741,
-0.22376314604679));
#4398=CARTESIAN_POINT('Ctrl Pts',(-1.09728268713976,-0.177024326825049,
-0.243890930799338));
#4399=CARTESIAN_POINT('Ctrl Pts',(-1.08664560412098,-0.227269801620063,
-0.287406530683753));
#4400=CARTESIAN_POINT('Ctrl Pts',(-1.0788165083757,-0.251265615809407,-0.316022600643821));
#4401=CARTESIAN_POINT('Ctrl Pts',(-1.06356957703048,-0.279889827963178,
-0.363699428370918));
#4402=CARTESIAN_POINT('Ctrl Pts',(-1.05494634094458,-0.290879136862659,
-0.388295406390235));
#4403=CARTESIAN_POINT('Ctrl Pts',(-1.03504317708586,-0.305251990234488,
-0.438600874831839));
#4404=CARTESIAN_POINT('Ctrl Pts',(-1.02374168767024,-0.308638795020976,
-0.46430090015576));
#4405=CARTESIAN_POINT('Ctrl Pts',(-1.00129756308006,-0.308638795020976,
-0.510906605094603));
#4406=CARTESIAN_POINT('Ctrl Pts',(-0.988250837578047,-0.305251990234488,
-0.535766169015486));
#4407=CARTESIAN_POINT('Ctrl Pts',(-0.961329858300736,-0.290879136862659,
-0.582692035672022));
#4408=CARTESIAN_POINT('Ctrl Pts',(-0.947476448101718,-0.279889827963178,
-0.604769294586516));
#4409=CARTESIAN_POINT('Ctrl Pts',(-0.919707509403859,-0.251265615809407,
-0.646415841396062));
#4410=CARTESIAN_POINT('Ctrl Pts',(-0.902215926359523,-0.227269801620064,
-0.670378702718353));
#4411=CARTESIAN_POINT('Ctrl Pts',(-0.87482617317514,-0.177024326825049,
-0.705826641853758));
#4412=CARTESIAN_POINT('Ctrl Pts',(-0.861652925570091,-0.144299303100741,
-0.721590372101268));
#4413=CARTESIAN_POINT('Ctrl Pts',(-0.848766861100456,-0.0928409665394229,
-0.736604687327351));
#4414=CARTESIAN_POINT('Ctrl Pts',(-0.84559647055299,-0.0762225747374255,
-0.740223768851063));
#4415=CARTESIAN_POINT('Ctrl Pts',(-0.843383895613249,-0.0595300000000001,
-0.742736168477219));
#4416=CARTESIAN_POINT('',(-0.536443649899847,-0.05953,-0.987512846410683));
#4417=CARTESIAN_POINT('Origin',(0.,-0.05953,0.));
#4418=CARTESIAN_POINT('',(0.0548532617164172,-0.05953,-1.12247250791415));
#4419=CARTESIAN_POINT('Ctrl Pts',(-0.536443649899848,-0.0595300000000001,
-0.987512846410683));
#4420=CARTESIAN_POINT('Ctrl Pts',(-0.533501897135712,-0.0762225747374254,
-0.989110885965947));
#4421=CARTESIAN_POINT('Ctrl Pts',(-0.529268075276156,-0.0928409665394227,
-0.991396466802469));
#4422=CARTESIAN_POINT('Ctrl Pts',(-0.511762781179147,-0.144299303100741,
-1.00061845128527));
#4423=CARTESIAN_POINT('Ctrl Pts',(-0.493462957200432,-0.177024326825049,
-1.0099536580922));
#4424=CARTESIAN_POINT('Ctrl Pts',(-0.45280897844858,-0.227269801620063,
-1.02876878445619));
#4425=CARTESIAN_POINT('Ctrl Pts',(-0.425554672694337,-0.251265615809407,
-1.04048957871266));
#4426=CARTESIAN_POINT('Ctrl Pts',(-0.3787731215897,-0.279889827963178,-1.05829506364875));
#4427=CARTESIAN_POINT('Ctrl Pts',(-0.354166711873529,-0.290879136862659,
-1.06688848765783));
#4428=CARTESIAN_POINT('Ctrl Pts',(-0.302426893214944,-0.305251990234488,
-1.08269251410343));
#4429=CARTESIAN_POINT('Ctrl Pts',(-0.275287440920027,-0.308638795020976,
-1.0898803575765));
#4430=CARTESIAN_POINT('Ctrl Pts',(-0.224855950742601,-0.308638795020976,
-1.10139101611326));
#4431=CARTESIAN_POINT('Ctrl Pts',(-0.19728546073067,-0.305251990234488,
-1.10669035995599));
#4432=CARTESIAN_POINT('Ctrl Pts',(-0.143812384801039,-0.290879136862659,
-1.11490049012186));
#4433=CARTESIAN_POINT('Ctrl Pts',(-0.117914228755037,-0.279889827963178,
-1.1178344036749));
#4434=CARTESIAN_POINT('Ctrl Pts',(-0.0680399972366989,-0.251265615809407,
-1.12208997038458));
#4435=CARTESIAN_POINT('Ctrl Pts',(-0.0383992541984084,-0.227269801620063,
-1.12335509974011));
#4436=CARTESIAN_POINT('Ctrl Pts',(0.00639229239215326,-0.177024326825049,
-1.12404235695137));
#4437=CARTESIAN_POINT('Ctrl Pts',(0.0269302585198977,-0.144299303100741,
-1.12357162229597));
#4438=CARTESIAN_POINT('Ctrl Pts',(0.04670325263426,-0.0928409665394228,
-1.12285816383385));
#4439=CARTESIAN_POINT('Ctrl Pts',(0.0515094706813703,-0.0762225747374255,
-1.12263591311425));
#4440=CARTESIAN_POINT('Ctrl Pts',(0.0548532617164176,-0.0595300000000001,
-1.12247250791414));
#4441=CARTESIAN_POINT('',(0.437601487681057,-0.05953,-1.03511272300331));
#4442=CARTESIAN_POINT('Origin',(0.,-0.05953,0.));
#4443=CARTESIAN_POINT('',(0.911784794170997,-0.05953,-0.656964154625313));
#4444=CARTESIAN_POINT('Ctrl Pts',(0.437601487681056,-0.0595300000000001,
-1.03511272300331));
#4445=CARTESIAN_POINT('Ctrl Pts',(0.440685038163619,-0.0762225747374255,
-1.03380912944435));
#4446=CARTESIAN_POINT('Ctrl Pts',(0.445111721969657,-0.0928409665394228,
-1.03192403056628));
#4447=CARTESIAN_POINT('Ctrl Pts',(0.463236132117164,-0.144299303100741,
-1.0239876538093));
#4448=CARTESIAN_POINT('Ctrl Pts',(0.481944444320713,-0.177024326825049,
-1.01550068154148));
#4449=CARTESIAN_POINT('Ctrl Pts',(0.522002043615455,-0.227269801620064,
-0.995447160474328));
#4450=CARTESIAN_POINT('Ctrl Pts',(0.548158511259203,-0.251265615809407,
-0.981446681891443));
#4451=CARTESIAN_POINT('Ctrl Pts',(0.591247219971725,-0.279889827963178,
-0.955972930713954));
#4452=CARTESIAN_POINT('Ctrl Pts',(0.613307674922609,-0.290879136862659,
-0.942092777160053));
#4453=CARTESIAN_POINT('Ctrl Pts',(0.657923009631182,-0.305251990234487,
-0.91149460735272));
#4454=CARTESIAN_POINT('Ctrl Pts',(0.680463863683393,-0.308638795020976,
-0.894757676234429));
#4455=CARTESIAN_POINT('Ctrl Pts',(0.720906778729542,-0.308638795020976,
-0.862505527716294));
#4456=CARTESIAN_POINT('Ctrl Pts',(0.742239891936899,-0.305251990234488,
-0.844254137480381));
#4457=CARTESIAN_POINT('Ctrl Pts',(0.781998747691872,-0.290879136862659,
-0.80756613568454));
#4458=CARTESIAN_POINT('Ctrl Pts',(0.800439809856112,-0.279889827963178,
-0.789147407129765));
#4459=CARTESIAN_POINT('Ctrl Pts',(0.834863020612702,-0.251265615809407,
-0.752807465209441));
#4460=CARTESIAN_POINT('Ctrl Pts',(0.854332839576145,-0.227269801620064,
-0.73042219438957));
#4461=CARTESIAN_POINT('Ctrl Pts',(0.882797231409153,-0.177024326825049,
-0.695831250979106));
#4462=CARTESIAN_POINT('Ctrl Pts',(0.895234408667242,-0.144299303100741,
-0.679480524217551));
#4463=CARTESIAN_POINT('Ctrl Pts',(0.907004864562642,-0.0928409665394228,
-0.663576540841106));
#4464=CARTESIAN_POINT('Ctrl Pts',(0.909827729890942,-0.0762225747374256,
-0.659680317203144));
#4465=CARTESIAN_POINT('Ctrl Pts',(0.911784794170998,-0.0595300000000001,
-0.656964154625312));
#4466=CARTESIAN_POINT('',(1.08212377959455,-0.05953,-0.303251606722892));
#4467=CARTESIAN_POINT('Origin',(0.,-0.05953,0.));
#4468=CARTESIAN_POINT('',(1.08212377959455,-0.05953,0.303251606722892));
#4469=CARTESIAN_POINT('Ctrl Pts',(1.08212377959455,-0.0595300000000001,
-0.303251606722892));
#4470=CARTESIAN_POINT('Ctrl Pts',(1.0830271513892,-0.0762225747374255,-0.300028012588062));
#4471=CARTESIAN_POINT('Ctrl Pts',(1.08431331394788,-0.0928409665394228,
-0.2953917518996));
#4472=CARTESIAN_POINT('Ctrl Pts',(1.08940878963422,-0.144299303100741,-0.276273267473431));
#4473=CARTESIAN_POINT('Ctrl Pts',(1.09443784939331,-0.177024326825049,-0.256354979351213));
#4474=CARTESIAN_POINT('Ctrl Pts',(1.10373487993589,-0.227269801620064,-0.212533521233765));
#4475=CARTESIAN_POINT('Ctrl Pts',(1.10909715583869,-0.251265615809407,-0.183354415742157));
#4476=CARTESIAN_POINT('Ctrl Pts',(1.1160463456491,-0.279889827963178,-0.133783682657561));
#4477=CARTESIAN_POINT('Ctrl Pts',(1.11894887330541,-0.290879136862659,-0.107881990270302));
#4478=CARTESIAN_POINT('Ctrl Pts',(1.12284346704144,-0.305251990234488,-0.0539226701638766));
#4479=CARTESIAN_POINT('Ctrl Pts',(1.123812,-0.308638795020976,-0.025864214957475));
#4480=CARTESIAN_POINT('Ctrl Pts',(1.123812,-0.308638795020976,0.025864214957475));
#4481=CARTESIAN_POINT('Ctrl Pts',(1.12284346704144,-0.305251990234488,0.0539226701638766));
#4482=CARTESIAN_POINT('Ctrl Pts',(1.11894887330541,-0.290879136862659,0.107881990270302));
#4483=CARTESIAN_POINT('Ctrl Pts',(1.1160463456491,-0.279889827963178,0.133783682657561));
#4484=CARTESIAN_POINT('Ctrl Pts',(1.10909715583869,-0.251265615809407,0.183354415742157));
#4485=CARTESIAN_POINT('Ctrl Pts',(1.10373487993589,-0.227269801620064,0.212533521233765));
#4486=CARTESIAN_POINT('Ctrl Pts',(1.09443784939331,-0.177024326825049,0.256354979351213));
#4487=CARTESIAN_POINT('Ctrl Pts',(1.08940878963422,-0.144299303100741,0.276273267473431));
#4488=CARTESIAN_POINT('Ctrl Pts',(1.08431331394788,-0.0928409665394228,
0.2953917518996));
#4489=CARTESIAN_POINT('Ctrl Pts',(1.0830271513892,-0.0762225747374255,0.300028012588062));
#4490=CARTESIAN_POINT('Ctrl Pts',(1.08212377959455,-0.0595300000000001,
0.303251606722892));
#4491=CARTESIAN_POINT('Origin',(0.,-0.05953,0.));
#4492=CARTESIAN_POINT('Origin',(0.,-0.05953,0.));
#4493=CARTESIAN_POINT('',(0.0589974094846122,-0.05953,1.07456964270265));
#4494=CARTESIAN_POINT('Origin',(0.,-0.05953,0.));
#4495=CARTESIAN_POINT('Origin',(-0.244773027351946,-0.05953,1.07242070340001));
#4496=CARTESIAN_POINT('Origin',(-0.244773027351946,0.,1.07242070340001));
#4497=CARTESIAN_POINT('',(-0.519393123750572,-0.05953,0.942555777842682));
#4498=CARTESIAN_POINT('Ctrl Pts',(-0.519393123750572,-0.05953,0.942555777842682));
#4499=CARTESIAN_POINT('Ctrl Pts',(-0.513714466572041,-0.0925528133349865,
0.945684988399766));
#4500=CARTESIAN_POINT('Ctrl Pts',(-0.503136848051455,-0.124911173756694,
0.951483858396181));
#4501=CARTESIAN_POINT('Ctrl Pts',(-0.47593627990192,-0.177924977804098,
0.965323333309091));
#4502=CARTESIAN_POINT('Ctrl Pts',(-0.460931856495794,-0.199697230012983,
0.972669835243841));
#4503=CARTESIAN_POINT('Ctrl Pts',(-0.426157505475872,-0.237895043532788,
0.988400002689705));
#4504=CARTESIAN_POINT('Ctrl Pts',(-0.406380688682952,-0.254319232363049,
0.996771768218699));
#4505=CARTESIAN_POINT('Ctrl Pts',(-0.364750145543744,-0.28018331644634,
1.01272583306292));
#4506=CARTESIAN_POINT('Ctrl Pts',(-0.340838910881557,-0.29104845371857,
1.02112815447116));
#4507=CARTESIAN_POINT('Ctrl Pts',(-0.290495481564827,-0.30527573347708,
1.036574285215));
#4508=CARTESIAN_POINT('Ctrl Pts',(-0.264056468041074,-0.308638795020976,
1.04359501395068));
#4509=CARTESIAN_POINT('Ctrl Pts',(-0.214892249704082,-0.308638795020976,
1.05481642595959));
#4510=CARTESIAN_POINT('Ctrl Pts',(-0.188025341585962,-0.30527573347708,
1.05996242598502));
#4511=CARTESIAN_POINT('Ctrl Pts',(-0.135965654106109,-0.29104845371857,
1.06788913840721));
#4512=CARTESIAN_POINT('Ctrl Pts',(-0.110776745452494,-0.28018331644634,
1.07069360430242));
#4513=CARTESIAN_POINT('Ctrl Pts',(-0.0663467128214646,-0.254319232363049,
1.07438230428002));
#4514=CARTESIAN_POINT('Ctrl Pts',(-0.0448960436540983,-0.237895043532788,
1.07542044338697));
#4515=CARTESIAN_POINT('Ctrl Pts',(-0.00674037211528124,-0.199697230012983,
1.07633607767727));
#4516=CARTESIAN_POINT('Ctrl Pts',(0.00996567398334777,-0.177924977804098,
1.07622728347683));
#4517=CARTESIAN_POINT('Ctrl Pts',(0.0404772621979741,-0.124911173756694,
1.07556023164702));
#4518=CARTESIAN_POINT('Ctrl Pts',(0.0525234025782719,-0.0925528133349865,
1.07492508698591));
#4519=CARTESIAN_POINT('Ctrl Pts',(0.0589974094846124,-0.05953,1.07456964270265));
#4520=CARTESIAN_POINT('Origin',(-0.244773027351946,-0.05953,1.07242070340001));
#4521=CARTESIAN_POINT('Origin',(0.,-0.05953,0.));
#4522=CARTESIAN_POINT('',(-0.803348093619616,-0.05953,0.716109245731214));
#4523=CARTESIAN_POINT('Origin',(0.,-0.05953,0.));
#4524=CARTESIAN_POINT('Origin',(-0.991065754692661,-0.05953,0.477272113029314));
#4525=CARTESIAN_POINT('Origin',(-0.991065754692661,0.,0.477272113029314));
#4526=CARTESIAN_POINT('',(-1.06075609691358,-0.05953,0.181596019242328));
#4527=CARTESIAN_POINT('Ctrl Pts',(-1.06075609691358,-0.05953,0.181596019242328));
#4528=CARTESIAN_POINT('Ctrl Pts',(-1.05966202740332,-0.0925528133349865,
0.187986803072856));
#4529=CARTESIAN_POINT('Ctrl Pts',(-1.05760072925372,-0.124911173756694,
0.199872254546857));
#4530=CARTESIAN_POINT('Ctrl Pts',(-1.05146158959546,-0.177924977804098,
0.22976728653846));
#4531=CARTESIAN_POINT('Ctrl Pts',(-1.04785021111757,-0.199697230012983,
0.246078686169301));
#4532=CARTESIAN_POINT('Ctrl Pts',(-1.03846709802406,-0.237895043532788,
0.283073967563097));
#4533=CARTESIAN_POINT('Ctrl Pts',(-1.03268176429485,-0.254319232363049,
0.303755815985685));
#4534=CARTESIAN_POINT('Ctrl Pts',(-1.01919893537026,-0.28018331644634,0.346251081972725));
#4535=CARTESIAN_POINT('Ctrl Pts',(-1.01085972381132,-0.29104845371857,0.370184399726282));
#4536=CARTESIAN_POINT('Ctrl Pts',(-0.99154738033959,-0.30527573347708,0.419174982698463));
#4537=CARTESIAN_POINT('Ctrl Pts',(-0.980551951791748,-0.308638795020976,
0.444223188605045));
#4538=CARTESIAN_POINT('Ctrl Pts',(-0.958671816228589,-0.308638795020976,
0.489657758261848));
#4539=CARTESIAN_POINT('Ctrl Pts',(-0.945943877838127,-0.30527573347708,
0.51387163140139));
#4540=CARTESIAN_POINT('Ctrl Pts',(-0.91968254693063,-0.29104845371857,0.559515758398093));
#4541=CARTESIAN_POINT('Ctrl Pts',(-0.906170138993533,-0.28018331644634,
0.580957796077825));
#4542=CARTESIAN_POINT('Ctrl Pts',(-0.8813524085237,-0.254319232363049,0.617994461173994));
#4543=CARTESIAN_POINT('Ctrl Pts',(-0.868789784891799,-0.237895043532788,
0.635412538795143));
#4544=CARTESIAN_POINT('Ctrl Pts',(-0.845715984518854,-0.199697230012983,
0.66581473268113));
#4545=CARTESIAN_POINT('Ctrl Pts',(-0.835214876415962,-0.177924977804098,
0.678808213394124));
#4546=CARTESIAN_POINT('Ctrl Pts',(-0.815669690204649,-0.124911173756694,
0.702247233627224));
#4547=CARTESIAN_POINT('Ctrl Pts',(-0.807662468433796,-0.0925528133349865,
0.711269279199861));
#4548=CARTESIAN_POINT('Ctrl Pts',(-0.803348093619616,-0.05953,0.716109245731214));
#4549=CARTESIAN_POINT('Origin',(-0.991065754692661,-0.05953,0.477272113029314));
#4550=CARTESIAN_POINT('Origin',(0.,-0.05953,0.));
#4551=CARTESIAN_POINT('',(-1.076188,-0.05953,1.31795018948079E-16));
#4552=CARTESIAN_POINT('Origin',(0.,-0.05953,0.));
#4553=CARTESIAN_POINT('',(-1.06075609691358,-0.05953,-0.181596019242328));
#4554=CARTESIAN_POINT('Origin',(0.,-0.05953,0.));
#4555=CARTESIAN_POINT('Origin',(-0.991065754692661,-0.05953,-0.477272113029314));
#4556=CARTESIAN_POINT('Origin',(-0.991065754692661,0.,-0.477272113029314));
#4557=CARTESIAN_POINT('',(-0.803348093619616,-0.05953,-0.716109245731215));
#4558=CARTESIAN_POINT('Ctrl Pts',(-0.803348093619616,-0.05953,-0.716109245731215));
#4559=CARTESIAN_POINT('Ctrl Pts',(-0.807662468433795,-0.0925528133349865,
-0.711269279199862));
#4560=CARTESIAN_POINT('Ctrl Pts',(-0.815669690204649,-0.124911173756694,
-0.702247233627224));
#4561=CARTESIAN_POINT('Ctrl Pts',(-0.835214876415962,-0.177924977804098,
-0.678808213394124));
#4562=CARTESIAN_POINT('Ctrl Pts',(-0.845715984518854,-0.199697230012983,
-0.66581473268113));
#4563=CARTESIAN_POINT('Ctrl Pts',(-0.868789784891799,-0.237895043532788,
-0.635412538795143));
#4564=CARTESIAN_POINT('Ctrl Pts',(-0.8813524085237,-0.254319232363049,-0.617994461173994));
#4565=CARTESIAN_POINT('Ctrl Pts',(-0.906170138993533,-0.28018331644634,
-0.580957796077826));
#4566=CARTESIAN_POINT('Ctrl Pts',(-0.91968254693063,-0.29104845371857,-0.559515758398093));
#4567=CARTESIAN_POINT('Ctrl Pts',(-0.945943877838127,-0.30527573347708,
-0.51387163140139));
#4568=CARTESIAN_POINT('Ctrl Pts',(-0.958671816228589,-0.308638795020976,
-0.489657758261848));
#4569=CARTESIAN_POINT('Ctrl Pts',(-0.980551951791748,-0.308638795020976,
-0.444223188605045));
#4570=CARTESIAN_POINT('Ctrl Pts',(-0.99154738033959,-0.30527573347708,-0.419174982698463));
#4571=CARTESIAN_POINT('Ctrl Pts',(-1.01085972381132,-0.29104845371857,-0.370184399726282));
#4572=CARTESIAN_POINT('Ctrl Pts',(-1.01919893537026,-0.28018331644634,-0.346251081972725));
#4573=CARTESIAN_POINT('Ctrl Pts',(-1.03268176429485,-0.254319232363049,
-0.303755815985685));
#4574=CARTESIAN_POINT('Ctrl Pts',(-1.03846709802406,-0.237895043532788,
-0.283073967563097));
#4575=CARTESIAN_POINT('Ctrl Pts',(-1.04785021111757,-0.199697230012983,
-0.246078686169302));
#4576=CARTESIAN_POINT('Ctrl Pts',(-1.05146158959546,-0.177924977804098,
-0.229767286538461));
#4577=CARTESIAN_POINT('Ctrl Pts',(-1.05760072925372,-0.124911173756694,
-0.199872254546858));
#4578=CARTESIAN_POINT('Ctrl Pts',(-1.05966202740332,-0.0925528133349864,
-0.187986803072857));
#4579=CARTESIAN_POINT('Ctrl Pts',(-1.06075609691358,-0.05953,-0.181596019242328));
#4580=CARTESIAN_POINT('Origin',(-0.991065754692661,-0.05953,-0.477272113029314));
#4581=CARTESIAN_POINT('Origin',(0.,-0.05953,0.));
#4582=CARTESIAN_POINT('',(-0.519393123750572,-0.05953,-0.942555777842682));
#4583=CARTESIAN_POINT('Origin',(0.,-0.05953,0.));
#4584=CARTESIAN_POINT('Origin',(-0.244773027351946,-0.05953,-1.07242070340001));
#4585=CARTESIAN_POINT('Origin',(-0.244773027351946,0.,-1.07242070340001));
#4586=CARTESIAN_POINT('',(0.0589974094846125,-0.05953,-1.07456964270265));
#4587=CARTESIAN_POINT('Ctrl Pts',(0.0589974094846127,-0.05953,-1.07456964270265));
#4588=CARTESIAN_POINT('Ctrl Pts',(0.0525234025782722,-0.0925528133349865,
-1.07492508698591));
#4589=CARTESIAN_POINT('Ctrl Pts',(0.0404772621979744,-0.124911173756694,
-1.07556023164702));
#4590=CARTESIAN_POINT('Ctrl Pts',(0.0099656739833481,-0.177924977804098,
-1.07622728347683));
#4591=CARTESIAN_POINT('Ctrl Pts',(-0.00674037211528096,-0.199697230012983,
-1.07633607767727));
#4592=CARTESIAN_POINT('Ctrl Pts',(-0.044896043654098,-0.237895043532788,
-1.07542044338697));
#4593=CARTESIAN_POINT('Ctrl Pts',(-0.0663467128214644,-0.254319232363049,
-1.07438230428002));
#4594=CARTESIAN_POINT('Ctrl Pts',(-0.110776745452493,-0.28018331644634,
-1.07069360430242));
#4595=CARTESIAN_POINT('Ctrl Pts',(-0.135965654106109,-0.29104845371857,
-1.06788913840721));
#4596=CARTESIAN_POINT('Ctrl Pts',(-0.188025341585962,-0.30527573347708,
-1.05996242598502));
#4597=CARTESIAN_POINT('Ctrl Pts',(-0.214892249704082,-0.308638795020976,
-1.05481642595959));
#4598=CARTESIAN_POINT('Ctrl Pts',(-0.264056468041074,-0.308638795020976,
-1.04359501395068));
#4599=CARTESIAN_POINT('Ctrl Pts',(-0.290495481564827,-0.30527573347708,
-1.036574285215));
#4600=CARTESIAN_POINT('Ctrl Pts',(-0.340838910881557,-0.291048453718569,
-1.02112815447116));
#4601=CARTESIAN_POINT('Ctrl Pts',(-0.364750145543744,-0.28018331644634,
-1.01272583306292));
#4602=CARTESIAN_POINT('Ctrl Pts',(-0.406380688682952,-0.254319232363049,
-0.996771768218699));
#4603=CARTESIAN_POINT('Ctrl Pts',(-0.426157505475872,-0.237895043532788,
-0.988400002689705));
#4604=CARTESIAN_POINT('Ctrl Pts',(-0.460931856495794,-0.199697230012983,
-0.972669835243841));
#4605=CARTESIAN_POINT('Ctrl Pts',(-0.475936279901919,-0.177924977804098,
-0.965323333309091));
#4606=CARTESIAN_POINT('Ctrl Pts',(-0.503136848051454,-0.124911173756694,
-0.951483858396181));
#4607=CARTESIAN_POINT('Ctrl Pts',(-0.513714466572041,-0.0925528133349865,
-0.945684988399766));
#4608=CARTESIAN_POINT('Ctrl Pts',(-0.519393123750572,-0.05953,-0.942555777842682));
#4609=CARTESIAN_POINT('Origin',(-0.244773027351946,-0.05953,-1.07242070340001));
#4610=CARTESIAN_POINT('Origin',(0.,-0.05953,0.));
#4611=CARTESIAN_POINT('',(0.413083465285518,-0.05953,-0.993751811093549));
#4612=CARTESIAN_POINT('Origin',(0.,-0.05953,0.));
#4613=CARTESIAN_POINT('Origin',(0.685838782044607,-0.05953,-0.860014630714833));
#4614=CARTESIAN_POINT('Origin',(0.685838782044607,0.,-0.860014630714833));
#4615=CARTESIAN_POINT('',(0.876916659919095,-0.05953,-0.623857181492959));
#4616=CARTESIAN_POINT('Ctrl Pts',(0.876916659919095,-0.05953,-0.623857181492958));
#4617=CARTESIAN_POINT('Ctrl Pts',(0.873158080166742,-0.0925528133349865,
-0.62914037979579));
#4618=CARTESIAN_POINT('Ctrl Pts',(0.866144010579847,-0.124911173756694,
-0.638954437806245));
#4619=CARTESIAN_POINT('Ctrl Pts',(0.847641868610495,-0.177924977804098,
-0.663225258065736));
#4620=CARTESIAN_POINT('Ctrl Pts',(0.837310877969633,-0.199697230012983,
-0.676354402927683));
#4621=CARTESIAN_POINT('Ctrl Pts',(0.81280533416753,-0.237895043532788,-0.705614819529209));
#4622=CARTESIAN_POINT('Ctrl Pts',(0.798619410861634,-0.254319232363049,
-0.721738358858166));
#4623=CARTESIAN_POINT('Ctrl Pts',(0.768033796848072,-0.28018331644634,-0.754175290318038));
#4624=CARTESIAN_POINT('Ctrl Pts',(0.750136149454208,-0.29104845371857,-0.772120216227122));
#4625=CARTESIAN_POINT('Ctrl Pts',(0.711480111898423,-0.30527573347708,-0.807879894508811));
#4626=CARTESIAN_POINT('Ctrl Pts',(0.690705563850638,-0.308638795020976,
-0.825676810575913));
#4627=CARTESIAN_POINT('Ctrl Pts',(0.651278921914856,-0.308638795020976,
-0.857118508332695));
#4628=CARTESIAN_POINT('Ctrl Pts',(0.629305439856167,-0.30527573347708,-0.873412008702649));
#4629=CARTESIAN_POINT('Ctrl Pts',(0.585840553788742,-0.29104845371857,-0.903141581680914));
#4630=CARTESIAN_POINT('Ctrl Pts',(0.564362943424239,-0.28018331644634,-0.916597376014514));
#4631=CARTESIAN_POINT('Ctrl Pts',(0.525933334162556,-0.254319232363049,
-0.939198248544427));
#4632=CARTESIAN_POINT('Ctrl Pts',(0.507057380724533,-0.237895043532788,
-0.949440676105255));
#4633=CARTESIAN_POINT('Ctrl Pts',(0.473077587363686,-0.199697230012983,
-0.966820759530997));
#4634=CARTESIAN_POINT('Ctrl Pts',(0.457978755888596,-0.177924977804098,
-0.973971221090534));
#4635=CARTESIAN_POINT('Ctrl Pts',(0.430199341854858,-0.124911173756694,
-0.986608710139579));
#4636=CARTESIAN_POINT('Ctrl Pts',(0.419070565453384,-0.0925528133349865,
-0.991263089003441));
#4637=CARTESIAN_POINT('Ctrl Pts',(0.413083465285518,-0.05953,-0.993751811093549));
#4638=CARTESIAN_POINT('Origin',(0.685838782044607,-0.05953,-0.860014630714833));
#4639=CARTESIAN_POINT('Origin',(0.,-0.208355,0.));
#4640=CARTESIAN_POINT('',(-1.076188,-0.35718,1.31795018948079E-16));
#4641=CARTESIAN_POINT('Origin',(0.,-0.35718,0.));
#4642=CARTESIAN_POINT('',(-1.076188,-0.208355,1.31795018948079E-16));
#4643=CARTESIAN_POINT('',(1.03449977959455,-0.05953,0.296632461748266));
#4644=CARTESIAN_POINT('Origin',(0.,-0.05953,0.));
#4645=CARTESIAN_POINT('',(1.03449977959455,-0.05953,-0.296632461748266));
#4646=CARTESIAN_POINT('Ctrl Pts',(1.03449977959455,-0.05953,0.296632461748267));
#4647=CARTESIAN_POINT('Ctrl Pts',(1.03628691421076,-0.0925528133349865,
0.290399865505497));
#4648=CARTESIAN_POINT('Ctrl Pts',(1.03958665287714,-0.124911173756694,0.278797079997872));
#4649=CARTESIAN_POINT('Ctrl Pts',(1.0470264474309,-0.177924977804098,0.249198913998601));
#4650=CARTESIAN_POINT('Ctrl Pts',(1.05084995891418,-0.199697230012983,0.232935932341942));
#4651=CARTESIAN_POINT('Ctrl Pts',(1.05844771715377,-0.237895043532788,0.195533155353269));
#4652=CARTESIAN_POINT('Ctrl Pts',(1.06220882929878,-0.254319232363049,0.17438929156337));
#4653=CARTESIAN_POINT('Ctrl Pts',(1.06849922508772,-0.28018331644634,0.130252399648131));
#4654=CARTESIAN_POINT('Ctrl Pts',(1.07137013248666,-0.29104845371857,0.105070977154072));
#4655=CARTESIAN_POINT('Ctrl Pts',(1.07522652957392,-0.30527573347708,0.0525526752791107));
#4656=CARTESIAN_POINT('Ctrl Pts',(1.076188,-0.308638795020976,0.025214283908933));
#4657=CARTESIAN_POINT('Ctrl Pts',(1.076188,-0.308638795020976,-0.025214283908933));
#4658=CARTESIAN_POINT('Ctrl Pts',(1.07522652957392,-0.30527573347708,-0.0525526752791107));
#4659=CARTESIAN_POINT('Ctrl Pts',(1.07137013248666,-0.29104845371857,-0.105070977154072));
#4660=CARTESIAN_POINT('Ctrl Pts',(1.06849922508772,-0.28018331644634,-0.130252399648131));
#4661=CARTESIAN_POINT('Ctrl Pts',(1.06220882929878,-0.254319232363049,-0.17438929156337));
#4662=CARTESIAN_POINT('Ctrl Pts',(1.05844771715377,-0.237895043532788,-0.195533155353269));
#4663=CARTESIAN_POINT('Ctrl Pts',(1.05084995891418,-0.199697230012983,-0.232935932341942));
#4664=CARTESIAN_POINT('Ctrl Pts',(1.0470264474309,-0.177924977804098,-0.249198913998601));
#4665=CARTESIAN_POINT('Ctrl Pts',(1.03958665287714,-0.124911173756694,-0.278797079997872));
#4666=CARTESIAN_POINT('Ctrl Pts',(1.03628691421076,-0.0925528133349865,
-0.290399865505497));
#4667=CARTESIAN_POINT('Ctrl Pts',(1.03449977959455,-0.05953,-0.296632461748267));
#4668=CARTESIAN_POINT('Origin',(0.,-0.05953,0.));
#4669=CARTESIAN_POINT('Origin',(0.,-0.05953,0.));
#4670=CARTESIAN_POINT('Origin',(1.1,-0.05953,0.));
#4671=CARTESIAN_POINT('Origin',(1.1,0.,0.));
#4672=CARTESIAN_POINT('Origin',(1.1,-0.05953,0.));
#4673=CARTESIAN_POINT('Origin',(0.,-0.35718,0.));
#4674=CARTESIAN_POINT('Origin',(0.,-0.05953,0.));
#4752=UNCERTAINTY_MEASURE_WITH_UNIT(LENGTH_MEASURE(0.001),#4778,
'DISTANCE_ACCURACY_VALUE',
'Maximum model space distance between geometric entities at asserted c
onnectivities');
#4755=UNCERTAINTY_MEASURE_WITH_UNIT(LENGTH_MEASURE(0.001),#4778,
'DISTANCE_ACCURACY_VALUE',
'Maximum model space distance between geometric entities at asserted c
onnectivities');
#4774=(
GEOMETRIC_REPRESENTATION_CONTEXT(3)
GLOBAL_UNCERTAINTY_ASSIGNED_CONTEXT((#4752))
GLOBAL_UNIT_ASSIGNED_CONTEXT((#4778,#4780,#4781))
REPRESENTATION_CONTEXT('','3D')
);
#4777=(
GEOMETRIC_REPRESENTATION_CONTEXT(3)
GLOBAL_UNCERTAINTY_ASSIGNED_CONTEXT((#4755))
GLOBAL_UNIT_ASSIGNED_CONTEXT((#4778,#4780,#4781))
REPRESENTATION_CONTEXT('','3D')
);
#4778=(
LENGTH_UNIT()
NAMED_UNIT(*)
SI_UNIT(.CENTI.,.METRE.)
);
#4780=(
NAMED_UNIT(*)
PLANE_ANGLE_UNIT()
SI_UNIT($,.RADIAN.)
);
#4781=(
NAMED_UNIT(*)
SI_UNIT($,.STERADIAN.)
SOLID_ANGLE_UNIT()
);
#4800=SHAPE_DEFINITION_REPRESENTATION(#4853,#4889);
#4853=PRODUCT_DEFINITION_SHAPE('',$,#4911);
#4889=SHAPE_REPRESENTATION('',(#2841),#4774);
#4892=PRODUCT_DEFINITION_CONTEXT('part definition',#4957,'design');
#4911=PRODUCT_DEFINITION('Cage','Cage',#4932,#4892);
#4932=PRODUCT_DEFINITION_FORMATION('',$,#4977);
#4957=APPLICATION_CONTEXT(
'Core Data for Automotive Mechanical Design Process');
#4958=PRODUCT_CONTEXT('part definition',#4957,'mechanical');
#4977=PRODUCT('Cage','Cage','Cage',(#4958));
#5050=COLOUR_RGB('Grey',0.48,0.52,0.57);
#5051=FILL_AREA_STYLE_COLOUR('',#5050);
#5052=FILL_AREA_STYLE('',(#5051));
#5053=SURFACE_STYLE_FILL_AREA(#5052);
#5054=SURFACE_SIDE_STYLE('',(#5053));
#5055=SURFACE_STYLE_USAGE(.BOTH.,#5054);
#5056=PRESENTATION_STYLE_ASSIGNMENT((#5055));
ENDSEC;
END-ISO-10303-21;
